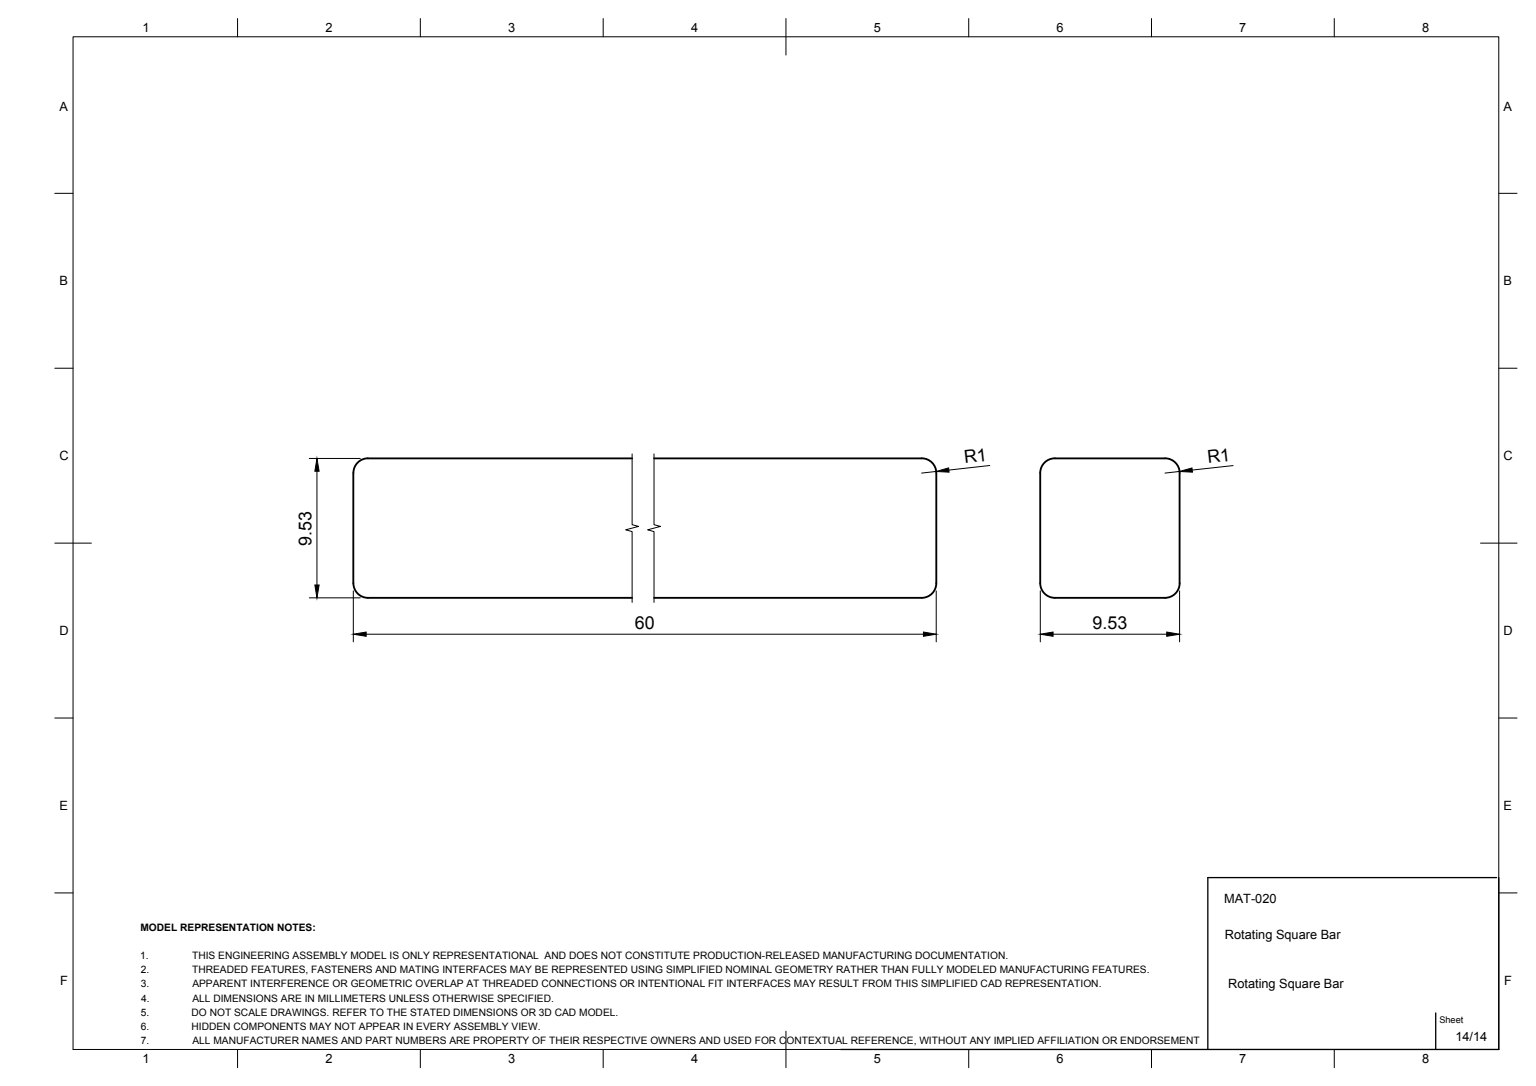
ISO-10303-21;
HEADER;
/* Generated by software containing ST-Developer
 * from STEP Tools, Inc. (www.steptools.com) 
 */

FILE_DESCRIPTION(
/* description */ ('STEP AP214'),
/* implementation_level */ '2;1');

FILE_NAME(
/* name */ 'Rotating Square Bar.step',
/* time_stamp */ '2026-11-14T06:20:50-08:00',
/* author */ (''),
/* organization */ (''),
/* preprocessor_version */ 'ST-DEVELOPER v20.2',
/* originating_system */ 'Autodesk Translation Framework v15.17.0.0',
/* authorisation */ '');

FILE_SCHEMA (('AUTOMOTIVE_DESIGN { 1 0 10303 214 3 1 1 }'));
ENDSEC;

DATA;
#10=MECHANICAL_DESIGN_GEOMETRIC_PRESENTATION_REPRESENTATION('',(#965),#20658);
#116=SPHERICAL_SURFACE('',#4025,1.);
#117=SPHERICAL_SURFACE('',#4028,1.);
#118=SPHERICAL_SURFACE('',#4045,1.);
#119=SPHERICAL_SURFACE('',#4047,1.);
#120=SPHERICAL_SURFACE('',#4049,1.);
#121=SPHERICAL_SURFACE('',#4051,1.);
#122=SPHERICAL_SURFACE('',#4061,1.);
#123=SPHERICAL_SURFACE('',#4063,1.);
#431=PLANE('',#4016);
#432=PLANE('',#4017);
#433=PLANE('',#4018);
#434=PLANE('',#4019);
#435=PLANE('',#4020);
#436=PLANE('',#4021);
#604=LINE('',#20388,#797);
#605=LINE('',#20390,#798);
#606=LINE('',#20392,#799);
#607=LINE('',#20393,#800);
#608=LINE('',#20397,#801);
#609=LINE('',#20399,#802);
#610=LINE('',#20401,#803);
#611=LINE('',#20402,#804);
#612=LINE('',#20406,#805);
#613=LINE('',#20408,#806);
#614=LINE('',#20410,#807);
#615=LINE('',#20411,#808);
#616=LINE('',#20415,#809);
#617=LINE('',#20417,#810);
#618=LINE('',#20419,#811);
#619=LINE('',#20420,#812);
#620=LINE('',#20424,#813);
#621=LINE('',#20426,#814);
#622=LINE('',#20428,#815);
#623=LINE('',#20429,#816);
#624=LINE('',#20433,#817);
#625=LINE('',#20435,#818);
#626=LINE('',#20437,#819);
#627=LINE('',#20438,#820);
#797=VECTOR('',#4727,1000.);
#798=VECTOR('',#4728,1000.);
#799=VECTOR('',#4729,1000.);
#800=VECTOR('',#4730,1000.);
#801=VECTOR('',#4733,1000.);
#802=VECTOR('',#4734,1000.);
#803=VECTOR('',#4735,1000.);
#804=VECTOR('',#4736,1000.);
#805=VECTOR('',#4739,1000.);
#806=VECTOR('',#4740,1000.);
#807=VECTOR('',#4741,1000.);
#808=VECTOR('',#4742,1000.);
#809=VECTOR('',#4745,1000.);
#810=VECTOR('',#4746,1000.);
#811=VECTOR('',#4747,1000.);
#812=VECTOR('',#4748,1000.);
#813=VECTOR('',#4751,1000.);
#814=VECTOR('',#4752,1000.);
#815=VECTOR('',#4753,1000.);
#816=VECTOR('',#4754,1000.);
#817=VECTOR('',#4757,1000.);
#818=VECTOR('',#4758,1000.);
#819=VECTOR('',#4759,1000.);
#820=VECTOR('',#4760,1000.);
#917=CYLINDRICAL_SURFACE('',#4022,1.);
#918=CYLINDRICAL_SURFACE('',#4031,1.);
#919=CYLINDRICAL_SURFACE('',#4033,1.);
#920=CYLINDRICAL_SURFACE('',#4035,1.);
#921=CYLINDRICAL_SURFACE('',#4038,1.);
#922=CYLINDRICAL_SURFACE('',#4040,1.);
#923=CYLINDRICAL_SURFACE('',#4042,1.);
#924=CYLINDRICAL_SURFACE('',#4053,1.);
#925=CYLINDRICAL_SURFACE('',#4055,1.);
#926=CYLINDRICAL_SURFACE('',#4057,1.);
#927=CYLINDRICAL_SURFACE('',#4059,1.);
#928=CYLINDRICAL_SURFACE('',#4065,1.);
#941=SHAPE_REPRESENTATION_RELATIONSHIP('SRR','None',#20725,#953);
#953=ADVANCED_BREP_SHAPE_REPRESENTATION('',(#977),#20655);
#965=STYLED_ITEM('',(#20786),#977);
#977=MANIFOLD_SOLID_BREP('Body1',#3660);
#1147=FACE_OUTER_BOUND('',#1379,.T.);
#1148=FACE_OUTER_BOUND('',#1380,.T.);
#1149=FACE_OUTER_BOUND('',#1381,.T.);
#1150=FACE_OUTER_BOUND('',#1382,.T.);
#1151=FACE_OUTER_BOUND('',#1383,.T.);
#1152=FACE_OUTER_BOUND('',#1384,.T.);
#1153=FACE_OUTER_BOUND('',#1385,.T.);
#1154=FACE_OUTER_BOUND('',#1386,.T.);
#1155=FACE_OUTER_BOUND('',#1387,.T.);
#1156=FACE_OUTER_BOUND('',#1388,.T.);
#1157=FACE_OUTER_BOUND('',#1389,.T.);
#1158=FACE_OUTER_BOUND('',#1390,.T.);
#1159=FACE_OUTER_BOUND('',#1391,.T.);
#1160=FACE_OUTER_BOUND('',#1392,.T.);
#1161=FACE_OUTER_BOUND('',#1393,.T.);
#1162=FACE_OUTER_BOUND('',#1394,.T.);
#1163=FACE_OUTER_BOUND('',#1395,.T.);
#1164=FACE_OUTER_BOUND('',#1396,.T.);
#1165=FACE_OUTER_BOUND('',#1397,.T.);
#1166=FACE_OUTER_BOUND('',#1398,.T.);
#1167=FACE_OUTER_BOUND('',#1399,.T.);
#1168=FACE_OUTER_BOUND('',#1400,.T.);
#1169=FACE_OUTER_BOUND('',#1401,.T.);
#1170=FACE_OUTER_BOUND('',#1402,.T.);
#1171=FACE_OUTER_BOUND('',#1403,.T.);
#1172=FACE_OUTER_BOUND('',#1404,.T.);
#1379=EDGE_LOOP('',(#3272,#3273,#3274,#3275));
#1380=EDGE_LOOP('',(#3276,#3277,#3278,#3279));
#1381=EDGE_LOOP('',(#3280,#3281,#3282,#3283));
#1382=EDGE_LOOP('',(#3284,#3285,#3286,#3287));
#1383=EDGE_LOOP('',(#3288,#3289,#3290,#3291));
#1384=EDGE_LOOP('',(#3292,#3293,#3294,#3295));
#1385=EDGE_LOOP('',(#3296,#3297,#3298,#3299));
#1386=EDGE_LOOP('',(#3300,#3301,#3302));
#1387=EDGE_LOOP('',(#3303,#3304,#3305));
#1388=EDGE_LOOP('',(#3306,#3307,#3308,#3309));
#1389=EDGE_LOOP('',(#3310,#3311,#3312,#3313));
#1390=EDGE_LOOP('',(#3314,#3315,#3316,#3317));
#1391=EDGE_LOOP('',(#3318,#3319,#3320,#3321));
#1392=EDGE_LOOP('',(#3322,#3323,#3324,#3325));
#1393=EDGE_LOOP('',(#3326,#3327,#3328,#3329));
#1394=EDGE_LOOP('',(#3330,#3331,#3332));
#1395=EDGE_LOOP('',(#3333,#3334,#3335));
#1396=EDGE_LOOP('',(#3336,#3337,#3338));
#1397=EDGE_LOOP('',(#3339,#3340,#3341));
#1398=EDGE_LOOP('',(#3342,#3343,#3344,#3345));
#1399=EDGE_LOOP('',(#3346,#3347,#3348,#3349));
#1400=EDGE_LOOP('',(#3350,#3351,#3352,#3353));
#1401=EDGE_LOOP('',(#3354,#3355,#3356,#3357));
#1402=EDGE_LOOP('',(#3358,#3359,#3360));
#1403=EDGE_LOOP('',(#3361,#3362,#3363));
#1404=EDGE_LOOP('',(#3364,#3365,#3366,#3367));
#1507=CIRCLE('',#4023,1.);
#1508=CIRCLE('',#4024,1.);
#1509=CIRCLE('',#4026,1.);
#1510=CIRCLE('',#4027,1.);
#1511=CIRCLE('',#4029,1.);
#1512=CIRCLE('',#4030,1.);
#1513=CIRCLE('',#4032,1.);
#1514=CIRCLE('',#4034,1.);
#1515=CIRCLE('',#4036,1.);
#1516=CIRCLE('',#4037,1.);
#1517=CIRCLE('',#4039,1.);
#1518=CIRCLE('',#4041,1.);
#1519=CIRCLE('',#4043,1.);
#1520=CIRCLE('',#4044,1.);
#1521=CIRCLE('',#4046,1.);
#1522=CIRCLE('',#4048,1.);
#1523=CIRCLE('',#4050,1.);
#1524=CIRCLE('',#4052,1.);
#1525=CIRCLE('',#4054,1.);
#1526=CIRCLE('',#4056,1.);
#1527=CIRCLE('',#4058,1.);
#1528=CIRCLE('',#4060,1.);
#1529=CIRCLE('',#4062,1.);
#1530=CIRCLE('',#4064,1.);
#1835=VERTEX_POINT('',#20386);
#1836=VERTEX_POINT('',#20387);
#1837=VERTEX_POINT('',#20389);
#1838=VERTEX_POINT('',#20391);
#1839=VERTEX_POINT('',#20395);
#1840=VERTEX_POINT('',#20396);
#1841=VERTEX_POINT('',#20398);
#1842=VERTEX_POINT('',#20400);
#1843=VERTEX_POINT('',#20404);
#1844=VERTEX_POINT('',#20405);
#1845=VERTEX_POINT('',#20407);
#1846=VERTEX_POINT('',#20409);
#1847=VERTEX_POINT('',#20413);
#1848=VERTEX_POINT('',#20414);
#1849=VERTEX_POINT('',#20416);
#1850=VERTEX_POINT('',#20418);
#1851=VERTEX_POINT('',#20422);
#1852=VERTEX_POINT('',#20423);
#1853=VERTEX_POINT('',#20425);
#1854=VERTEX_POINT('',#20427);
#1855=VERTEX_POINT('',#20431);
#1856=VERTEX_POINT('',#20432);
#1857=VERTEX_POINT('',#20434);
#1858=VERTEX_POINT('',#20436);
#2318=EDGE_CURVE('',#1835,#1836,#604,.T.);
#2319=EDGE_CURVE('',#1836,#1837,#605,.T.);
#2320=EDGE_CURVE('',#1837,#1838,#606,.T.);
#2321=EDGE_CURVE('',#1838,#1835,#607,.T.);
#2322=EDGE_CURVE('',#1839,#1840,#608,.T.);
#2323=EDGE_CURVE('',#1840,#1841,#609,.T.);
#2324=EDGE_CURVE('',#1841,#1842,#610,.T.);
#2325=EDGE_CURVE('',#1842,#1839,#611,.T.);
#2326=EDGE_CURVE('',#1843,#1844,#612,.T.);
#2327=EDGE_CURVE('',#1844,#1845,#613,.T.);
#2328=EDGE_CURVE('',#1845,#1846,#614,.T.);
#2329=EDGE_CURVE('',#1846,#1843,#615,.T.);
#2330=EDGE_CURVE('',#1847,#1848,#616,.T.);
#2331=EDGE_CURVE('',#1848,#1849,#617,.T.);
#2332=EDGE_CURVE('',#1849,#1850,#618,.T.);
#2333=EDGE_CURVE('',#1850,#1847,#619,.T.);
#2334=EDGE_CURVE('',#1851,#1852,#620,.T.);
#2335=EDGE_CURVE('',#1852,#1853,#621,.T.);
#2336=EDGE_CURVE('',#1853,#1854,#622,.T.);
#2337=EDGE_CURVE('',#1854,#1851,#623,.T.);
#2338=EDGE_CURVE('',#1855,#1856,#624,.T.);
#2339=EDGE_CURVE('',#1856,#1857,#625,.T.);
#2340=EDGE_CURVE('',#1857,#1858,#626,.T.);
#2341=EDGE_CURVE('',#1858,#1855,#627,.T.);
#2342=EDGE_CURVE('',#1842,#1843,#1507,.T.);
#2343=EDGE_CURVE('',#1844,#1841,#1508,.T.);
#2344=EDGE_CURVE('',#1842,#1851,#1509,.T.);
#2345=EDGE_CURVE('',#1851,#1843,#1510,.T.);
#2346=EDGE_CURVE('',#1844,#1856,#1511,.T.);
#2347=EDGE_CURVE('',#1856,#1841,#1512,.T.);
#2348=EDGE_CURVE('',#1852,#1846,#1513,.T.);
#2349=EDGE_CURVE('',#1839,#1854,#1514,.T.);
#2350=EDGE_CURVE('',#1840,#1837,#1515,.T.);
#2351=EDGE_CURVE('',#1838,#1839,#1516,.T.);
#2352=EDGE_CURVE('',#1857,#1840,#1517,.T.);
#2353=EDGE_CURVE('',#1845,#1855,#1518,.T.);
#2354=EDGE_CURVE('',#1846,#1847,#1519,.T.);
#2355=EDGE_CURVE('',#1848,#1845,#1520,.T.);
#2356=EDGE_CURVE('',#1852,#1847,#1521,.T.);
#2357=EDGE_CURVE('',#1838,#1854,#1522,.T.);
#2358=EDGE_CURVE('',#1857,#1837,#1523,.T.);
#2359=EDGE_CURVE('',#1848,#1855,#1524,.T.);
#2360=EDGE_CURVE('',#1853,#1850,#1525,.T.);
#2361=EDGE_CURVE('',#1835,#1853,#1526,.T.);
#2362=EDGE_CURVE('',#1858,#1836,#1527,.T.);
#2363=EDGE_CURVE('',#1849,#1858,#1528,.T.);
#2364=EDGE_CURVE('',#1835,#1850,#1529,.T.);
#2365=EDGE_CURVE('',#1849,#1836,#1530,.T.);
#3272=ORIENTED_EDGE('',*,*,#2318,.T.);
#3273=ORIENTED_EDGE('',*,*,#2319,.T.);
#3274=ORIENTED_EDGE('',*,*,#2320,.T.);
#3275=ORIENTED_EDGE('',*,*,#2321,.T.);
#3276=ORIENTED_EDGE('',*,*,#2322,.T.);
#3277=ORIENTED_EDGE('',*,*,#2323,.T.);
#3278=ORIENTED_EDGE('',*,*,#2324,.T.);
#3279=ORIENTED_EDGE('',*,*,#2325,.T.);
#3280=ORIENTED_EDGE('',*,*,#2326,.T.);
#3281=ORIENTED_EDGE('',*,*,#2327,.T.);
#3282=ORIENTED_EDGE('',*,*,#2328,.T.);
#3283=ORIENTED_EDGE('',*,*,#2329,.T.);
#3284=ORIENTED_EDGE('',*,*,#2330,.T.);
#3285=ORIENTED_EDGE('',*,*,#2331,.T.);
#3286=ORIENTED_EDGE('',*,*,#2332,.T.);
#3287=ORIENTED_EDGE('',*,*,#2333,.T.);
#3288=ORIENTED_EDGE('',*,*,#2334,.T.);
#3289=ORIENTED_EDGE('',*,*,#2335,.T.);
#3290=ORIENTED_EDGE('',*,*,#2336,.T.);
#3291=ORIENTED_EDGE('',*,*,#2337,.T.);
#3292=ORIENTED_EDGE('',*,*,#2338,.T.);
#3293=ORIENTED_EDGE('',*,*,#2339,.T.);
#3294=ORIENTED_EDGE('',*,*,#2340,.T.);
#3295=ORIENTED_EDGE('',*,*,#2341,.T.);
#3296=ORIENTED_EDGE('',*,*,#2342,.F.);
#3297=ORIENTED_EDGE('',*,*,#2324,.F.);
#3298=ORIENTED_EDGE('',*,*,#2343,.F.);
#3299=ORIENTED_EDGE('',*,*,#2326,.F.);
#3300=ORIENTED_EDGE('',*,*,#2344,.F.);
#3301=ORIENTED_EDGE('',*,*,#2342,.T.);
#3302=ORIENTED_EDGE('',*,*,#2345,.F.);
#3303=ORIENTED_EDGE('',*,*,#2346,.F.);
#3304=ORIENTED_EDGE('',*,*,#2343,.T.);
#3305=ORIENTED_EDGE('',*,*,#2347,.F.);
#3306=ORIENTED_EDGE('',*,*,#2345,.T.);
#3307=ORIENTED_EDGE('',*,*,#2329,.F.);
#3308=ORIENTED_EDGE('',*,*,#2348,.F.);
#3309=ORIENTED_EDGE('',*,*,#2334,.F.);
#3310=ORIENTED_EDGE('',*,*,#2344,.T.);
#3311=ORIENTED_EDGE('',*,*,#2337,.F.);
#3312=ORIENTED_EDGE('',*,*,#2349,.F.);
#3313=ORIENTED_EDGE('',*,*,#2325,.F.);
#3314=ORIENTED_EDGE('',*,*,#2350,.F.);
#3315=ORIENTED_EDGE('',*,*,#2322,.F.);
#3316=ORIENTED_EDGE('',*,*,#2351,.F.);
#3317=ORIENTED_EDGE('',*,*,#2320,.F.);
#3318=ORIENTED_EDGE('',*,*,#2347,.T.);
#3319=ORIENTED_EDGE('',*,*,#2323,.F.);
#3320=ORIENTED_EDGE('',*,*,#2352,.F.);
#3321=ORIENTED_EDGE('',*,*,#2339,.F.);
#3322=ORIENTED_EDGE('',*,*,#2346,.T.);
#3323=ORIENTED_EDGE('',*,*,#2338,.F.);
#3324=ORIENTED_EDGE('',*,*,#2353,.F.);
#3325=ORIENTED_EDGE('',*,*,#2327,.F.);
#3326=ORIENTED_EDGE('',*,*,#2354,.F.);
#3327=ORIENTED_EDGE('',*,*,#2328,.F.);
#3328=ORIENTED_EDGE('',*,*,#2355,.F.);
#3329=ORIENTED_EDGE('',*,*,#2330,.F.);
#3330=ORIENTED_EDGE('',*,*,#2348,.T.);
#3331=ORIENTED_EDGE('',*,*,#2354,.T.);
#3332=ORIENTED_EDGE('',*,*,#2356,.F.);
#3333=ORIENTED_EDGE('',*,*,#2351,.T.);
#3334=ORIENTED_EDGE('',*,*,#2349,.T.);
#3335=ORIENTED_EDGE('',*,*,#2357,.F.);
#3336=ORIENTED_EDGE('',*,*,#2352,.T.);
#3337=ORIENTED_EDGE('',*,*,#2350,.T.);
#3338=ORIENTED_EDGE('',*,*,#2358,.F.);
#3339=ORIENTED_EDGE('',*,*,#2355,.T.);
#3340=ORIENTED_EDGE('',*,*,#2353,.T.);
#3341=ORIENTED_EDGE('',*,*,#2359,.F.);
#3342=ORIENTED_EDGE('',*,*,#2356,.T.);
#3343=ORIENTED_EDGE('',*,*,#2333,.F.);
#3344=ORIENTED_EDGE('',*,*,#2360,.F.);
#3345=ORIENTED_EDGE('',*,*,#2335,.F.);
#3346=ORIENTED_EDGE('',*,*,#2357,.T.);
#3347=ORIENTED_EDGE('',*,*,#2336,.F.);
#3348=ORIENTED_EDGE('',*,*,#2361,.F.);
#3349=ORIENTED_EDGE('',*,*,#2321,.F.);
#3350=ORIENTED_EDGE('',*,*,#2358,.T.);
#3351=ORIENTED_EDGE('',*,*,#2319,.F.);
#3352=ORIENTED_EDGE('',*,*,#2362,.F.);
#3353=ORIENTED_EDGE('',*,*,#2340,.F.);
#3354=ORIENTED_EDGE('',*,*,#2359,.T.);
#3355=ORIENTED_EDGE('',*,*,#2341,.F.);
#3356=ORIENTED_EDGE('',*,*,#2363,.F.);
#3357=ORIENTED_EDGE('',*,*,#2331,.F.);
#3358=ORIENTED_EDGE('',*,*,#2361,.T.);
#3359=ORIENTED_EDGE('',*,*,#2360,.T.);
#3360=ORIENTED_EDGE('',*,*,#2364,.F.);
#3361=ORIENTED_EDGE('',*,*,#2363,.T.);
#3362=ORIENTED_EDGE('',*,*,#2362,.T.);
#3363=ORIENTED_EDGE('',*,*,#2365,.F.);
#3364=ORIENTED_EDGE('',*,*,#2364,.T.);
#3365=ORIENTED_EDGE('',*,*,#2332,.F.);
#3366=ORIENTED_EDGE('',*,*,#2365,.T.);
#3367=ORIENTED_EDGE('',*,*,#2318,.F.);
#3609=ADVANCED_FACE('',(#1147),#431,.F.);
#3610=ADVANCED_FACE('',(#1148),#432,.F.);
#3611=ADVANCED_FACE('',(#1149),#433,.F.);
#3612=ADVANCED_FACE('',(#1150),#434,.F.);
#3613=ADVANCED_FACE('',(#1151),#435,.F.);
#3614=ADVANCED_FACE('',(#1152),#436,.T.);
#3615=ADVANCED_FACE('',(#1153),#917,.T.);
#3616=ADVANCED_FACE('',(#1154),#116,.T.);
#3617=ADVANCED_FACE('',(#1155),#117,.T.);
#3618=ADVANCED_FACE('',(#1156),#918,.T.);
#3619=ADVANCED_FACE('',(#1157),#919,.T.);
#3620=ADVANCED_FACE('',(#1158),#920,.T.);
#3621=ADVANCED_FACE('',(#1159),#921,.T.);
#3622=ADVANCED_FACE('',(#1160),#922,.T.);
#3623=ADVANCED_FACE('',(#1161),#923,.T.);
#3624=ADVANCED_FACE('',(#1162),#118,.T.);
#3625=ADVANCED_FACE('',(#1163),#119,.T.);
#3626=ADVANCED_FACE('',(#1164),#120,.T.);
#3627=ADVANCED_FACE('',(#1165),#121,.T.);
#3628=ADVANCED_FACE('',(#1166),#924,.T.);
#3629=ADVANCED_FACE('',(#1167),#925,.T.);
#3630=ADVANCED_FACE('',(#1168),#926,.T.);
#3631=ADVANCED_FACE('',(#1169),#927,.T.);
#3632=ADVANCED_FACE('',(#1170),#122,.T.);
#3633=ADVANCED_FACE('',(#1171),#123,.T.);
#3634=ADVANCED_FACE('',(#1172),#928,.T.);
#3660=CLOSED_SHELL('',(#3609,#3610,#3611,#3612,#3613,#3614,#3615,#3616,
#3617,#3618,#3619,#3620,#3621,#3622,#3623,#3624,#3625,#3626,#3627,#3628,
#3629,#3630,#3631,#3632,#3633,#3634));
#4015=AXIS2_PLACEMENT_3D('',#20384,#4723,#4724);
#4016=AXIS2_PLACEMENT_3D('',#20385,#4725,#4726);
#4017=AXIS2_PLACEMENT_3D('',#20394,#4731,#4732);
#4018=AXIS2_PLACEMENT_3D('',#20403,#4737,#4738);
#4019=AXIS2_PLACEMENT_3D('',#20412,#4743,#4744);
#4020=AXIS2_PLACEMENT_3D('',#20421,#4749,#4750);
#4021=AXIS2_PLACEMENT_3D('',#20430,#4755,#4756);
#4022=AXIS2_PLACEMENT_3D('',#20439,#4761,#4762);
#4023=AXIS2_PLACEMENT_3D('',#20440,#4763,#4764);
#4024=AXIS2_PLACEMENT_3D('',#20441,#4765,#4766);
#4025=AXIS2_PLACEMENT_3D('',#20442,#4767,#4768);
#4026=AXIS2_PLACEMENT_3D('',#20443,#4769,#4770);
#4027=AXIS2_PLACEMENT_3D('',#20444,#4771,#4772);
#4028=AXIS2_PLACEMENT_3D('',#20445,#4773,#4774);
#4029=AXIS2_PLACEMENT_3D('',#20446,#4775,#4776);
#4030=AXIS2_PLACEMENT_3D('',#20447,#4777,#4778);
#4031=AXIS2_PLACEMENT_3D('',#20448,#4779,#4780);
#4032=AXIS2_PLACEMENT_3D('',#20449,#4781,#4782);
#4033=AXIS2_PLACEMENT_3D('',#20450,#4783,#4784);
#4034=AXIS2_PLACEMENT_3D('',#20451,#4785,#4786);
#4035=AXIS2_PLACEMENT_3D('',#20452,#4787,#4788);
#4036=AXIS2_PLACEMENT_3D('',#20453,#4789,#4790);
#4037=AXIS2_PLACEMENT_3D('',#20454,#4791,#4792);
#4038=AXIS2_PLACEMENT_3D('',#20455,#4793,#4794);
#4039=AXIS2_PLACEMENT_3D('',#20456,#4795,#4796);
#4040=AXIS2_PLACEMENT_3D('',#20457,#4797,#4798);
#4041=AXIS2_PLACEMENT_3D('',#20458,#4799,#4800);
#4042=AXIS2_PLACEMENT_3D('',#20459,#4801,#4802);
#4043=AXIS2_PLACEMENT_3D('',#20460,#4803,#4804);
#4044=AXIS2_PLACEMENT_3D('',#20461,#4805,#4806);
#4045=AXIS2_PLACEMENT_3D('',#20462,#4807,#4808);
#4046=AXIS2_PLACEMENT_3D('',#20463,#4809,#4810);
#4047=AXIS2_PLACEMENT_3D('',#20464,#4811,#4812);
#4048=AXIS2_PLACEMENT_3D('',#20465,#4813,#4814);
#4049=AXIS2_PLACEMENT_3D('',#20466,#4815,#4816);
#4050=AXIS2_PLACEMENT_3D('',#20467,#4817,#4818);
#4051=AXIS2_PLACEMENT_3D('',#20468,#4819,#4820);
#4052=AXIS2_PLACEMENT_3D('',#20469,#4821,#4822);
#4053=AXIS2_PLACEMENT_3D('',#20470,#4823,#4824);
#4054=AXIS2_PLACEMENT_3D('',#20471,#4825,#4826);
#4055=AXIS2_PLACEMENT_3D('',#20472,#4827,#4828);
#4056=AXIS2_PLACEMENT_3D('',#20473,#4829,#4830);
#4057=AXIS2_PLACEMENT_3D('',#20474,#4831,#4832);
#4058=AXIS2_PLACEMENT_3D('',#20475,#4833,#4834);
#4059=AXIS2_PLACEMENT_3D('',#20476,#4835,#4836);
#4060=AXIS2_PLACEMENT_3D('',#20477,#4837,#4838);
#4061=AXIS2_PLACEMENT_3D('',#20478,#4839,#4840);
#4062=AXIS2_PLACEMENT_3D('',#20479,#4841,#4842);
#4063=AXIS2_PLACEMENT_3D('',#20480,#4843,#4844);
#4064=AXIS2_PLACEMENT_3D('',#20481,#4845,#4846);
#4065=AXIS2_PLACEMENT_3D('',#20482,#4847,#4848);
#4723=DIRECTION('axis',(0.,0.,1.));
#4724=DIRECTION('refdir',(1.,0.,0.));
#4725=DIRECTION('center_axis',(-1.,0.,0.));
#4726=DIRECTION('ref_axis',(0.,0.,1.));
#4727=DIRECTION('',(0.,-1.,0.));
#4728=DIRECTION('',(0.,0.,-1.));
#4729=DIRECTION('',(0.,1.,0.));
#4730=DIRECTION('',(0.,0.,1.));
#4731=DIRECTION('center_axis',(0.,0.,1.));
#4732=DIRECTION('ref_axis',(1.,0.,0.));
#4733=DIRECTION('',(0.,-1.,0.));
#4734=DIRECTION('',(-1.,0.,0.));
#4735=DIRECTION('',(0.,1.,0.));
#4736=DIRECTION('',(1.,0.,0.));
#4737=DIRECTION('center_axis',(1.,0.,0.));
#4738=DIRECTION('ref_axis',(0.,0.,-1.));
#4739=DIRECTION('',(0.,-1.,0.));
#4740=DIRECTION('',(0.,0.,1.));
#4741=DIRECTION('',(0.,1.,0.));
#4742=DIRECTION('',(0.,0.,-1.));
#4743=DIRECTION('center_axis',(0.,0.,-1.));
#4744=DIRECTION('ref_axis',(-1.,0.,0.));
#4745=DIRECTION('',(0.,-1.,0.));
#4746=DIRECTION('',(1.,0.,0.));
#4747=DIRECTION('',(0.,1.,0.));
#4748=DIRECTION('',(-1.,0.,0.));
#4749=DIRECTION('center_axis',(0.,-1.,0.));
#4750=DIRECTION('ref_axis',(0.,0.,-1.));
#4751=DIRECTION('',(0.,0.,1.));
#4752=DIRECTION('',(1.,0.,0.));
#4753=DIRECTION('',(0.,0.,-1.));
#4754=DIRECTION('',(-1.,0.,0.));
#4755=DIRECTION('center_axis',(0.,-1.,0.));
#4756=DIRECTION('ref_axis',(0.,0.,-1.));
#4757=DIRECTION('',(0.,0.,-1.));
#4758=DIRECTION('',(1.,0.,0.));
#4759=DIRECTION('',(0.,0.,1.));
#4760=DIRECTION('',(-1.,0.,0.));
#4761=DIRECTION('center_axis',(0.,-1.,0.));
#4762=DIRECTION('ref_axis',(0.,0.,-1.));
#4763=DIRECTION('center_axis',(0.,1.,0.));
#4764=DIRECTION('ref_axis',(0.,0.,1.));
#4765=DIRECTION('center_axis',(0.,-1.,0.));
#4766=DIRECTION('ref_axis',(0.,0.,-1.));
#4767=DIRECTION('center_axis',(0.,1.,0.));
#4768=DIRECTION('ref_axis',(0.,0.,1.));
#4769=DIRECTION('center_axis',(1.,0.,0.));
#4770=DIRECTION('ref_axis',(0.,0.,1.));
#4771=DIRECTION('center_axis',(0.,-8.67361737988404E-16,1.));
#4772=DIRECTION('ref_axis',(0.,1.,8.67361737988404E-16));
#4773=DIRECTION('center_axis',(1.,0.,0.));
#4774=DIRECTION('ref_axis',(0.,1.,-8.88178419700125E-16));
#4775=DIRECTION('center_axis',(-8.67361737988403E-16,0.,1.));
#4776=DIRECTION('ref_axis',(-1.,0.,-8.67361737988403E-16));
#4777=DIRECTION('center_axis',(1.,0.,0.));
#4778=DIRECTION('ref_axis',(0.,0.,1.));
#4779=DIRECTION('center_axis',(0.,0.,1.));
#4780=DIRECTION('ref_axis',(1.,0.,0.));
#4781=DIRECTION('center_axis',(0.,0.,1.));
#4782=DIRECTION('ref_axis',(1.,0.,0.));
#4783=DIRECTION('center_axis',(-1.,0.,0.));
#4784=DIRECTION('ref_axis',(0.,0.,1.));
#4785=DIRECTION('center_axis',(1.,0.,0.));
#4786=DIRECTION('ref_axis',(0.,0.,-1.));
#4787=DIRECTION('center_axis',(0.,-1.,0.));
#4788=DIRECTION('ref_axis',(0.,0.,-1.));
#4789=DIRECTION('center_axis',(0.,-1.,0.));
#4790=DIRECTION('ref_axis',(0.,0.,-1.));
#4791=DIRECTION('center_axis',(0.,1.,0.));
#4792=DIRECTION('ref_axis',(0.,0.,1.));
#4793=DIRECTION('center_axis',(1.,0.,0.));
#4794=DIRECTION('ref_axis',(0.,0.,-1.));
#4795=DIRECTION('center_axis',(1.,0.,0.));
#4796=DIRECTION('ref_axis',(0.,0.,-1.));
#4797=DIRECTION('center_axis',(0.,0.,-1.));
#4798=DIRECTION('ref_axis',(-1.,0.,0.));
#4799=DIRECTION('center_axis',(0.,0.,1.));
#4800=DIRECTION('ref_axis',(1.,0.,0.));
#4801=DIRECTION('center_axis',(0.,-1.,0.));
#4802=DIRECTION('ref_axis',(0.,0.,-1.));
#4803=DIRECTION('center_axis',(0.,1.,0.));
#4804=DIRECTION('ref_axis',(0.,0.,1.));
#4805=DIRECTION('center_axis',(0.,-1.,0.));
#4806=DIRECTION('ref_axis',(0.,0.,-1.));
#4807=DIRECTION('center_axis',(0.,1.,0.));
#4808=DIRECTION('ref_axis',(0.,0.,1.));
#4809=DIRECTION('center_axis',(1.,0.,0.));
#4810=DIRECTION('ref_axis',(0.,0.,1.));
#4811=DIRECTION('center_axis',(0.,1.,0.));
#4812=DIRECTION('ref_axis',(-1.,0.,0.));
#4813=DIRECTION('center_axis',(0.,0.,1.));
#4814=DIRECTION('ref_axis',(-1.,0.,0.));
#4815=DIRECTION('center_axis',(1.,0.,0.));
#4816=DIRECTION('ref_axis',(0.,1.,-8.88178419700125E-16));
#4817=DIRECTION('center_axis',(0.,0.,1.));
#4818=DIRECTION('ref_axis',(-1.,0.,0.));
#4819=DIRECTION('center_axis',(0.,0.,1.));
#4820=DIRECTION('ref_axis',(0.,-1.,0.));
#4821=DIRECTION('center_axis',(1.,0.,0.));
#4822=DIRECTION('ref_axis',(0.,0.,1.));
#4823=DIRECTION('center_axis',(1.,0.,0.));
#4824=DIRECTION('ref_axis',(0.,0.,-1.));
#4825=DIRECTION('center_axis',(1.,0.,0.));
#4826=DIRECTION('ref_axis',(0.,0.,-1.));
#4827=DIRECTION('center_axis',(0.,0.,-1.));
#4828=DIRECTION('ref_axis',(-1.,0.,0.));
#4829=DIRECTION('center_axis',(0.,0.,1.));
#4830=DIRECTION('ref_axis',(1.,0.,0.));
#4831=DIRECTION('center_axis',(0.,0.,1.));
#4832=DIRECTION('ref_axis',(1.,0.,0.));
#4833=DIRECTION('center_axis',(0.,0.,1.));
#4834=DIRECTION('ref_axis',(1.,0.,0.));
#4835=DIRECTION('center_axis',(-1.,0.,0.));
#4836=DIRECTION('ref_axis',(0.,0.,1.));
#4837=DIRECTION('center_axis',(1.,0.,0.));
#4838=DIRECTION('ref_axis',(0.,0.,-1.));
#4839=DIRECTION('center_axis',(1.,0.,0.));
#4840=DIRECTION('ref_axis',(0.,0.,1.));
#4841=DIRECTION('center_axis',(0.,-1.,0.));
#4842=DIRECTION('ref_axis',(0.,0.,1.));
#4843=DIRECTION('center_axis',(1.,0.,0.));
#4844=DIRECTION('ref_axis',(0.,0.,-1.));
#4845=DIRECTION('center_axis',(0.,1.,0.));
#4846=DIRECTION('ref_axis',(0.,0.,-1.));
#4847=DIRECTION('center_axis',(0.,-1.,0.));
#4848=DIRECTION('ref_axis',(0.,0.,-1.));
#20384=CARTESIAN_POINT('',(0.,0.,0.));
#20385=CARTESIAN_POINT('Origin',(30.,9.53,4.7625));
#20386=CARTESIAN_POINT('',(30.,8.53,3.7625));
#20387=CARTESIAN_POINT('',(30.,1.,3.7625));
#20388=CARTESIAN_POINT('',(30.,9.53,3.7625));
#20389=CARTESIAN_POINT('',(30.,1.,-3.7625));
#20390=CARTESIAN_POINT('',(30.,1.,-4.7625));
#20391=CARTESIAN_POINT('',(30.,8.53,-3.7625));
#20392=CARTESIAN_POINT('',(30.,9.53,-3.7625));
#20393=CARTESIAN_POINT('',(30.,8.53,4.7625));
#20394=CARTESIAN_POINT('Origin',(-30.,9.53,-4.7625));
#20395=CARTESIAN_POINT('',(29.,8.53,-4.7625));
#20396=CARTESIAN_POINT('',(29.,1.,-4.7625));
#20397=CARTESIAN_POINT('',(29.,9.53,-4.7625));
#20398=CARTESIAN_POINT('',(-29.,1.,-4.7625));
#20399=CARTESIAN_POINT('',(-30.,1.,-4.7625));
#20400=CARTESIAN_POINT('',(-29.,8.53,-4.7625));
#20401=CARTESIAN_POINT('',(-29.,9.53,-4.7625));
#20402=CARTESIAN_POINT('',(-30.,8.53,-4.7625));
#20403=CARTESIAN_POINT('Origin',(-30.,9.53,4.7625));
#20404=CARTESIAN_POINT('',(-30.,8.53,-3.7625));
#20405=CARTESIAN_POINT('',(-30.,1.,-3.7625));
#20406=CARTESIAN_POINT('',(-30.,9.53,-3.7625));
#20407=CARTESIAN_POINT('',(-30.,1.,3.7625));
#20408=CARTESIAN_POINT('',(-30.,1.,4.7625));
#20409=CARTESIAN_POINT('',(-30.,8.53,3.7625));
#20410=CARTESIAN_POINT('',(-30.,9.53,3.7625));
#20411=CARTESIAN_POINT('',(-30.,8.53,4.7625));
#20412=CARTESIAN_POINT('Origin',(-30.,9.53,4.7625));
#20413=CARTESIAN_POINT('',(-29.,8.53,4.7625));
#20414=CARTESIAN_POINT('',(-29.,1.,4.7625));
#20415=CARTESIAN_POINT('',(-29.,9.53,4.7625));
#20416=CARTESIAN_POINT('',(29.,1.,4.7625));
#20417=CARTESIAN_POINT('',(30.,1.,4.7625));
#20418=CARTESIAN_POINT('',(29.,8.53,4.7625));
#20419=CARTESIAN_POINT('',(29.,9.53,4.7625));
#20420=CARTESIAN_POINT('',(-30.,8.53,4.7625));
#20421=CARTESIAN_POINT('Origin',(0.,9.53,0.));
#20422=CARTESIAN_POINT('',(-29.,9.53,-3.7625));
#20423=CARTESIAN_POINT('',(-29.,9.53,3.7625));
#20424=CARTESIAN_POINT('',(-29.,9.53,0.));
#20425=CARTESIAN_POINT('',(29.,9.53,3.7625));
#20426=CARTESIAN_POINT('',(0.,9.53,3.7625));
#20427=CARTESIAN_POINT('',(29.,9.53,-3.7625));
#20428=CARTESIAN_POINT('',(29.,9.53,0.));
#20429=CARTESIAN_POINT('',(0.,9.53,-3.7625));
#20430=CARTESIAN_POINT('Origin',(0.,0.,0.));
#20431=CARTESIAN_POINT('',(-29.,0.,3.7625));
#20432=CARTESIAN_POINT('',(-29.,0.,-3.7625));
#20433=CARTESIAN_POINT('',(-29.,0.,-4.7625));
#20434=CARTESIAN_POINT('',(29.,0.,-3.7625));
#20435=CARTESIAN_POINT('',(30.,0.,-3.7625));
#20436=CARTESIAN_POINT('',(29.,0.,3.7625));
#20437=CARTESIAN_POINT('',(29.,0.,4.7625));
#20438=CARTESIAN_POINT('',(-30.,0.,3.7625));
#20439=CARTESIAN_POINT('Origin',(-29.,9.53,-3.7625));
#20440=CARTESIAN_POINT('Origin',(-29.,8.53,-3.7625));
#20441=CARTESIAN_POINT('Origin',(-29.,1.,-3.7625));
#20442=CARTESIAN_POINT('Origin',(-29.,8.53,-3.7625));
#20443=CARTESIAN_POINT('Origin',(-29.,8.53,-3.7625));
#20444=CARTESIAN_POINT('Origin',(-29.,8.53,-3.7625));
#20445=CARTESIAN_POINT('Origin',(-29.,1.,-3.7625));
#20446=CARTESIAN_POINT('Origin',(-29.,1.,-3.7625));
#20447=CARTESIAN_POINT('Origin',(-29.,1.,-3.7625));
#20448=CARTESIAN_POINT('Origin',(-29.,8.53,0.));
#20449=CARTESIAN_POINT('Origin',(-29.,8.53,3.7625));
#20450=CARTESIAN_POINT('Origin',(0.,8.53,-3.7625));
#20451=CARTESIAN_POINT('Origin',(29.,8.53,-3.7625));
#20452=CARTESIAN_POINT('Origin',(29.,9.53,-3.7625));
#20453=CARTESIAN_POINT('Origin',(29.,1.,-3.7625));
#20454=CARTESIAN_POINT('Origin',(29.,8.53,-3.7625));
#20455=CARTESIAN_POINT('Origin',(-30.,1.,-3.7625));
#20456=CARTESIAN_POINT('Origin',(29.,1.,-3.7625));
#20457=CARTESIAN_POINT('Origin',(-29.,1.,4.7625));
#20458=CARTESIAN_POINT('Origin',(-29.,1.,3.7625));
#20459=CARTESIAN_POINT('Origin',(-29.,9.53,3.7625));
#20460=CARTESIAN_POINT('Origin',(-29.,8.53,3.7625));
#20461=CARTESIAN_POINT('Origin',(-29.,1.,3.7625));
#20462=CARTESIAN_POINT('Origin',(-29.,8.53,3.7625));
#20463=CARTESIAN_POINT('Origin',(-29.,8.53,3.7625));
#20464=CARTESIAN_POINT('Origin',(29.,8.53,-3.7625));
#20465=CARTESIAN_POINT('Origin',(29.,8.53,-3.7625));
#20466=CARTESIAN_POINT('Origin',(29.,1.,-3.7625));
#20467=CARTESIAN_POINT('Origin',(29.,1.,-3.7625));
#20468=CARTESIAN_POINT('Origin',(-29.,1.,3.7625));
#20469=CARTESIAN_POINT('Origin',(-29.,1.,3.7625));
#20470=CARTESIAN_POINT('Origin',(0.,8.53,3.7625));
#20471=CARTESIAN_POINT('Origin',(29.,8.53,3.7625));
#20472=CARTESIAN_POINT('Origin',(29.,8.53,0.));
#20473=CARTESIAN_POINT('Origin',(29.,8.53,3.7625));
#20474=CARTESIAN_POINT('Origin',(29.,1.,4.7625));
#20475=CARTESIAN_POINT('Origin',(29.,1.,3.7625));
#20476=CARTESIAN_POINT('Origin',(-30.,1.,3.7625));
#20477=CARTESIAN_POINT('Origin',(29.,1.,3.7625));
#20478=CARTESIAN_POINT('Origin',(29.,8.53,3.7625));
#20479=CARTESIAN_POINT('Origin',(29.,8.53,3.7625));
#20480=CARTESIAN_POINT('Origin',(29.,1.,3.7625));
#20481=CARTESIAN_POINT('Origin',(29.,1.,3.7625));
#20482=CARTESIAN_POINT('Origin',(29.,9.53,3.7625));
#20641=UNCERTAINTY_MEASURE_WITH_UNIT(LENGTH_MEASURE(0.01),#20659,
'DISTANCE_ACCURACY_VALUE',
'Maximum model space distance between geometric entities at asserted c
onnectivities');
#20644=UNCERTAINTY_MEASURE_WITH_UNIT(LENGTH_MEASURE(0.01),#20659,
'DISTANCE_ACCURACY_VALUE',
'Maximum model space distance between geometric entities at asserted c
onnectivities');
#20655=(
GEOMETRIC_REPRESENTATION_CONTEXT(3)
GLOBAL_UNCERTAINTY_ASSIGNED_CONTEXT((#20641))
GLOBAL_UNIT_ASSIGNED_CONTEXT((#20659,#20661,#20662))
REPRESENTATION_CONTEXT('','3D')
);
#20658=(
GEOMETRIC_REPRESENTATION_CONTEXT(3)
GLOBAL_UNCERTAINTY_ASSIGNED_CONTEXT((#20644))
GLOBAL_UNIT_ASSIGNED_CONTEXT((#20659,#20661,#20662))
REPRESENTATION_CONTEXT('','3D')
);
#20659=(
LENGTH_UNIT()
NAMED_UNIT(*)
SI_UNIT(.MILLI.,.METRE.)
);
#20661=(
NAMED_UNIT(*)
PLANE_ANGLE_UNIT()
SI_UNIT($,.RADIAN.)
);
#20662=(
NAMED_UNIT(*)
SI_UNIT($,.STERADIAN.)
SOLID_ANGLE_UNIT()
);
#20673=SHAPE_DEFINITION_REPRESENTATION(#20686,#20725);
#20686=PRODUCT_DEFINITION_SHAPE('',$,#20739);
#20725=SHAPE_REPRESENTATION('',(#4015),#20655);
#20728=PRODUCT_DEFINITION_CONTEXT('part definition',#20769,'design');
#20739=PRODUCT_DEFINITION('Rotating Square Bar','Rotating Square Bar',#20752,
#20728);
#20752=PRODUCT_DEFINITION_FORMATION('',$,#20781);
#20769=APPLICATION_CONTEXT(
'Core Data for Automotive Mechanical Design Process');
#20770=PRODUCT_CONTEXT('part definition',#20769,'mechanical');
#20781=PRODUCT('Rotating Square Bar','Rotating Square Bar',$,(#20770));
#20786=PRESENTATION_STYLE_ASSIGNMENT((#20791));
#20791=SURFACE_STYLE_USAGE(.BOTH.,#20796);
#20796=SURFACE_SIDE_STYLE('',(#20801));
#20801=SURFACE_STYLE_FILL_AREA(#20806);
#20806=FILL_AREA_STYLE('Opaque(61,176,222)',(#20811));
#20811=FILL_AREA_STYLE_COLOUR('Opaque(61,176,222)',#20816);
#20816=COLOUR_RGB('Opaque(61,176,222)',0.23921568627451,0.690196078431373,
0.870588235294118);
ENDSEC;
END-ISO-10303-21;
